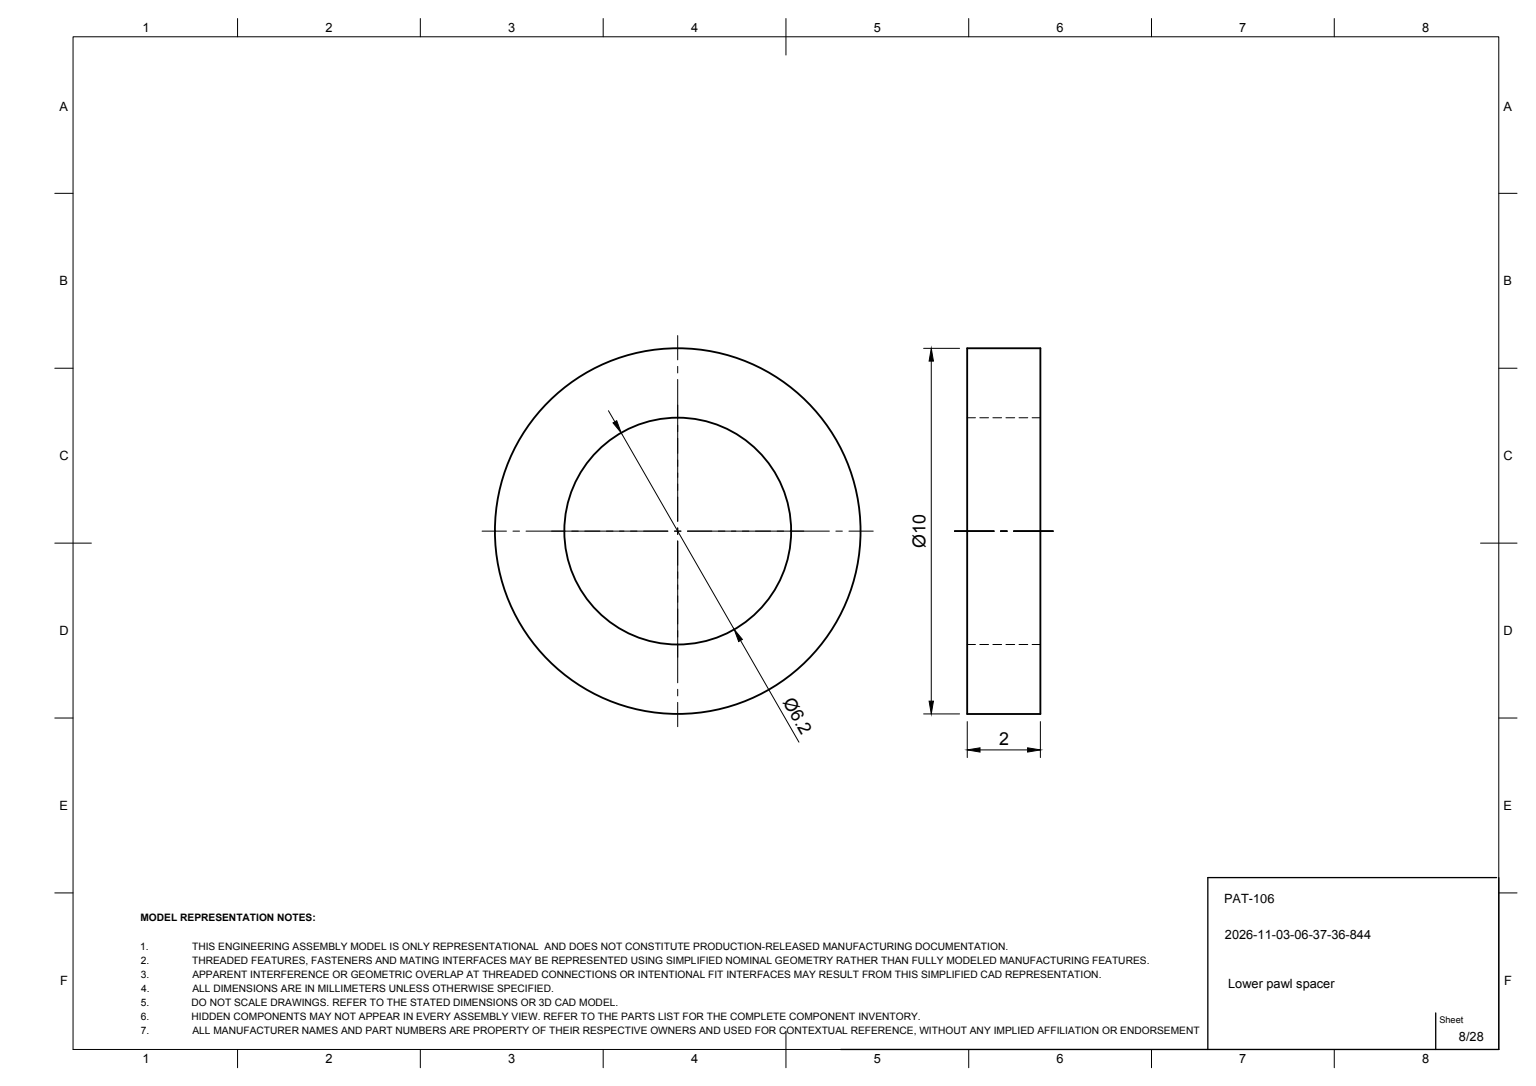
ISO-10303-21;
HEADER;
/* Generated by software containing ST-Developer
 * from STEP Tools, Inc. (www.steptools.com) 
 */

FILE_DESCRIPTION(
/* description */ ('Torsion-spring ratchet demonstrator'),
/* implementation_level */ '2;1');

FILE_NAME(
/* name */ 'Lower pawl spacer.step',
/* time_stamp */ '2026-10-29T17:29:17-07:00',
/* author */ (''),
/* organization */ (''),
/* preprocessor_version */ 'ST-DEVELOPER v20.2',
/* originating_system */ 'Autodesk Translation Framework v15.17.0.0',
/* authorisation */ '');

FILE_SCHEMA (('AUTOMOTIVE_DESIGN { 1 0 10303 214 3 1 1 }'));
ENDSEC;

DATA;
#10=MECHANICAL_DESIGN_GEOMETRIC_PRESENTATION_REPRESENTATION('',(#286),#11258);
#238=SHAPE_REPRESENTATION_RELATIONSHIP('SRR','None',#11364,#262);
#262=ADVANCED_BREP_SHAPE_REPRESENTATION('',(#318),#11234);
#286=STYLED_ITEM('',(#11598),#318);
#318=MANIFOLD_SOLID_BREP('Body1',#5157);
#369=FACE_BOUND('',#988,.T.);
#370=FACE_BOUND('',#990,.T.);
#455=PLANE('',#5528);
#456=PLANE('',#5529);
#656=FACE_OUTER_BOUND('',#985,.T.);
#657=FACE_OUTER_BOUND('',#986,.T.);
#658=FACE_OUTER_BOUND('',#987,.T.);
#659=FACE_OUTER_BOUND('',#989,.T.);
#985=EDGE_LOOP('',(#3580,#3581,#3582,#3583));
#986=EDGE_LOOP('',(#3584,#3585,#3586,#3587));
#987=EDGE_LOOP('',(#3588));
#988=EDGE_LOOP('',(#3589));
#989=EDGE_LOOP('',(#3590));
#990=EDGE_LOOP('',(#3591));
#1364=LINE('',#7833,#1747);
#1365=LINE('',#7839,#1748);
#1747=VECTOR('',#6247,0.31);
#1748=VECTOR('',#6254,0.5);
#2121=CIRCLE('',#5523,0.31);
#2122=CIRCLE('',#5524,0.31);
#2123=CIRCLE('',#5526,0.5);
#2124=CIRCLE('',#5527,0.5);
#2381=VERTEX_POINT('',#7830);
#2382=VERTEX_POINT('',#7832);
#2383=VERTEX_POINT('',#7836);
#2384=VERTEX_POINT('',#7838);
#2850=EDGE_CURVE('',#2381,#2381,#2121,.T.);
#2851=EDGE_CURVE('',#2381,#2382,#1364,.T.);
#2852=EDGE_CURVE('',#2382,#2382,#2122,.T.);
#2853=EDGE_CURVE('',#2383,#2383,#2123,.T.);
#2854=EDGE_CURVE('',#2383,#2384,#1365,.T.);
#2855=EDGE_CURVE('',#2384,#2384,#2124,.T.);
#3580=ORIENTED_EDGE('',*,*,#2850,.F.);
#3581=ORIENTED_EDGE('',*,*,#2851,.T.);
#3582=ORIENTED_EDGE('',*,*,#2852,.T.);
#3583=ORIENTED_EDGE('',*,*,#2851,.F.);
#3584=ORIENTED_EDGE('',*,*,#2853,.F.);
#3585=ORIENTED_EDGE('',*,*,#2854,.T.);
#3586=ORIENTED_EDGE('',*,*,#2855,.T.);
#3587=ORIENTED_EDGE('',*,*,#2854,.F.);
#3588=ORIENTED_EDGE('',*,*,#2853,.T.);
#3589=ORIENTED_EDGE('',*,*,#2850,.T.);
#3590=ORIENTED_EDGE('',*,*,#2855,.F.);
#3591=ORIENTED_EDGE('',*,*,#2852,.F.);
#4779=CYLINDRICAL_SURFACE('',#5522,0.31);
#4780=CYLINDRICAL_SURFACE('',#5525,0.5);
#4882=ADVANCED_FACE('',(#656),#4779,.F.);
#4883=ADVANCED_FACE('',(#657),#4780,.T.);
#4884=ADVANCED_FACE('',(#658,#369),#455,.T.);
#4885=ADVANCED_FACE('',(#659,#370),#456,.F.);
#5157=CLOSED_SHELL('',(#4882,#4883,#4884,#4885));
#5521=AXIS2_PLACEMENT_3D('',#7828,#6241,#6242);
#5522=AXIS2_PLACEMENT_3D('',#7829,#6243,#6244);
#5523=AXIS2_PLACEMENT_3D('',#7831,#6245,#6246);
#5524=AXIS2_PLACEMENT_3D('',#7834,#6248,#6249);
#5525=AXIS2_PLACEMENT_3D('',#7835,#6250,#6251);
#5526=AXIS2_PLACEMENT_3D('',#7837,#6252,#6253);
#5527=AXIS2_PLACEMENT_3D('',#7840,#6255,#6256);
#5528=AXIS2_PLACEMENT_3D('',#7841,#6257,#6258);
#5529=AXIS2_PLACEMENT_3D('',#7842,#6259,#6260);
#6241=DIRECTION('axis',(0.,0.,1.));
#6242=DIRECTION('refdir',(1.,0.,0.));
#6243=DIRECTION('center_axis',(0.,0.,1.));
#6244=DIRECTION('ref_axis',(1.,0.,0.));
#6245=DIRECTION('center_axis',(0.,0.,-1.));
#6246=DIRECTION('ref_axis',(1.,0.,0.));
#6247=DIRECTION('',(0.,0.,-1.));
#6248=DIRECTION('center_axis',(0.,0.,-1.));
#6249=DIRECTION('ref_axis',(1.,0.,0.));
#6250=DIRECTION('center_axis',(0.,0.,1.));
#6251=DIRECTION('ref_axis',(1.,0.,0.));
#6252=DIRECTION('center_axis',(0.,0.,1.));
#6253=DIRECTION('ref_axis',(1.,0.,0.));
#6254=DIRECTION('',(0.,0.,-1.));
#6255=DIRECTION('center_axis',(0.,0.,1.));
#6256=DIRECTION('ref_axis',(1.,0.,0.));
#6257=DIRECTION('center_axis',(0.,0.,1.));
#6258=DIRECTION('ref_axis',(1.,0.,0.));
#6259=DIRECTION('center_axis',(0.,0.,1.));
#6260=DIRECTION('ref_axis',(1.,0.,0.));
#7828=CARTESIAN_POINT('',(0.,0.,0.));
#7829=CARTESIAN_POINT('Origin',(6.5,-3.47,4.6));
#7830=CARTESIAN_POINT('',(6.19,-3.47,4.8));
#7831=CARTESIAN_POINT('Origin',(6.5,-3.47,4.8));
#7832=CARTESIAN_POINT('',(6.19,-3.47,4.6));
#7833=CARTESIAN_POINT('',(6.19,-3.47,4.6));
#7834=CARTESIAN_POINT('Origin',(6.5,-3.47,4.6));
#7835=CARTESIAN_POINT('Origin',(6.5,-3.47,4.6));
#7836=CARTESIAN_POINT('',(6.,-3.47,4.8));
#7837=CARTESIAN_POINT('Origin',(6.5,-3.47,4.8));
#7838=CARTESIAN_POINT('',(6.,-3.47,4.6));
#7839=CARTESIAN_POINT('',(6.,-3.47,4.6));
#7840=CARTESIAN_POINT('Origin',(6.5,-3.47,4.6));
#7841=CARTESIAN_POINT('Origin',(6.5,-3.47,4.8));
#7842=CARTESIAN_POINT('Origin',(6.5,-3.47,4.6));
#11204=UNCERTAINTY_MEASURE_WITH_UNIT(LENGTH_MEASURE(0.001),#11259,
'DISTANCE_ACCURACY_VALUE',
'Maximum model space distance between geometric entities at asserted c
onnectivities');
#11228=UNCERTAINTY_MEASURE_WITH_UNIT(LENGTH_MEASURE(0.001),#11259,
'DISTANCE_ACCURACY_VALUE',
'Maximum model space distance between geometric entities at asserted c
onnectivities');
#11234=(
GEOMETRIC_REPRESENTATION_CONTEXT(3)
GLOBAL_UNCERTAINTY_ASSIGNED_CONTEXT((#11204))
GLOBAL_UNIT_ASSIGNED_CONTEXT((#11259,#11261,#11262))
REPRESENTATION_CONTEXT('','3D')
);
#11258=(
GEOMETRIC_REPRESENTATION_CONTEXT(3)
GLOBAL_UNCERTAINTY_ASSIGNED_CONTEXT((#11228))
GLOBAL_UNIT_ASSIGNED_CONTEXT((#11259,#11261,#11262))
REPRESENTATION_CONTEXT('','3D')
);
#11259=(
LENGTH_UNIT()
NAMED_UNIT(*)
SI_UNIT(.CENTI.,.METRE.)
);
#11261=(
NAMED_UNIT(*)
PLANE_ANGLE_UNIT()
SI_UNIT($,.RADIAN.)
);
#11262=(
NAMED_UNIT(*)
SI_UNIT($,.STERADIAN.)
SOLID_ANGLE_UNIT()
);
#11268=SHAPE_DEFINITION_REPRESENTATION(#11297,#11364);
#11297=PRODUCT_DEFINITION_SHAPE('',$,#11394);
#11364=SHAPE_REPRESENTATION('',(#5521),#11234);
#11388=PRODUCT_DEFINITION_CONTEXT('part definition',#11477,'design');
#11394=PRODUCT_DEFINITION('Lower pawl spacer','Lower pawl spacer',#11423,
#11388);
#11423=PRODUCT_DEFINITION_FORMATION('',$,#11484);
#11477=APPLICATION_CONTEXT(
'Core Data for Automotive Mechanical Design Process');
#11478=PRODUCT_CONTEXT('part definition',#11477,'mechanical');
#11484=PRODUCT('Lower pawl spacer','Lower pawl spacer',
'Lower pawl spacer',(#11478));
#11592=COLOUR_RGB('Off White',0.89,0.88,0.83);
#11593=FILL_AREA_STYLE_COLOUR('',#11592);
#11594=FILL_AREA_STYLE('',(#11593));
#11595=SURFACE_STYLE_FILL_AREA(#11594);
#11596=SURFACE_SIDE_STYLE('',(#11595));
#11597=SURFACE_STYLE_USAGE(.BOTH.,#11596);
#11598=PRESENTATION_STYLE_ASSIGNMENT((#11597));
ENDSEC;
END-ISO-10303-21;
